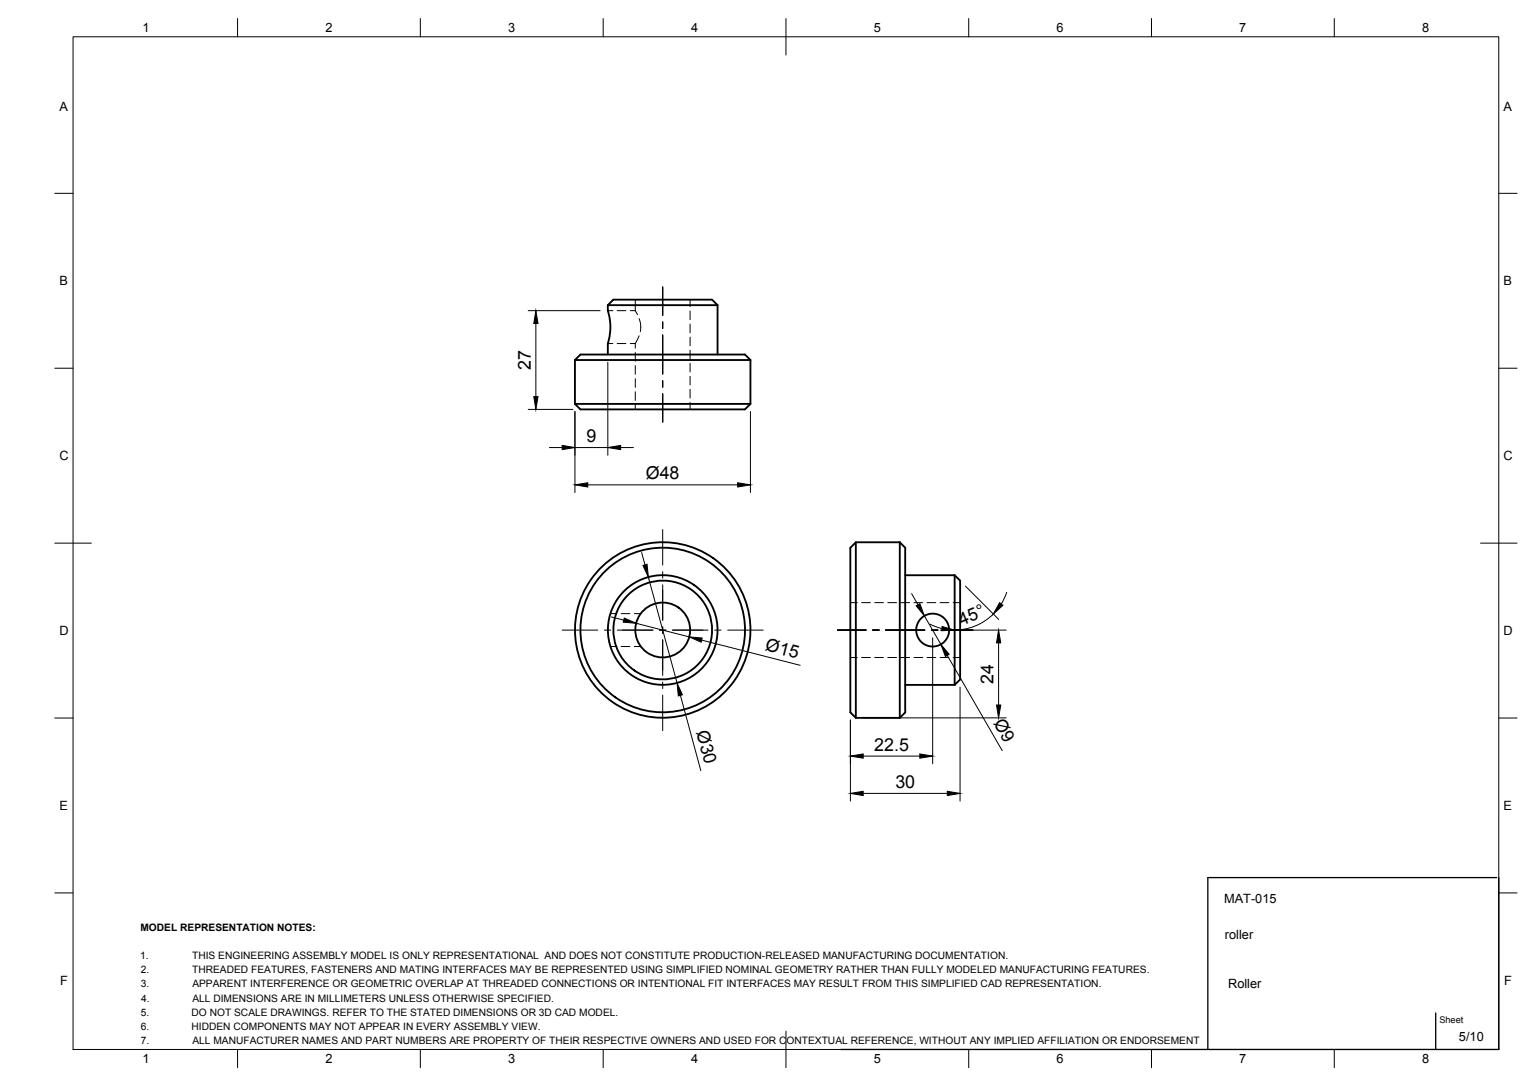
ISO-10303-21;
HEADER;
/* Generated by software containing ST-Developer
 * from STEP Tools, Inc. (www.steptools.com) 
 */

FILE_DESCRIPTION(
/* description */ ('STEP AP214'),
/* implementation_level */ '2;1');

FILE_NAME(
/* name */ 'Roller.step',
/* time_stamp */ '2026-11-14T06:03:18-08:00',
/* author */ (''),
/* organization */ (''),
/* preprocessor_version */ 'ST-DEVELOPER v20.2',
/* originating_system */ 'Autodesk Translation Framework v15.17.0.0',
/* authorisation */ '');

FILE_SCHEMA (('AUTOMOTIVE_DESIGN { 1 0 10303 214 3 1 1 }'));
ENDSEC;

DATA;
#10=MECHANICAL_DESIGN_GEOMETRIC_PRESENTATION_REPRESENTATION('',(#73),#3206);
#47=B_SPLINE_CURVE_WITH_KNOTS('',3,(#2691,#2692,#2693,#2694,#2695,#2696,
#2697,#2698,#2699,#2700,#2701,#2702,#2703,#2704,#2705,#2706,#2707,#2708),
 .UNSPECIFIED.,.F.,.F.,(4,2,2,2,2,2,2,2,4),(-1.36519473470625,-1.19451997041109,
-1.02384520611593,-0.853221286734528,-0.682597367353127,-0.511973447971726,
-0.341349528590325,-0.170674764295162,0.),.UNSPECIFIED.);
#48=B_SPLINE_CURVE_WITH_KNOTS('',3,(#2712,#2713,#2714,#2715,#2716,#2717,
#2718,#2719,#2720,#2721,#2722,#2723,#2724,#2725,#2726,#2727,#2728,#2729),
 .UNSPECIFIED.,.F.,.F.,(4,2,2,2,2,2,2,2,4),(-1.39899108486948,-1.22355122072177,
-1.04811135657406,-0.873803449504402,-0.699495542434742,-0.525187635365083,
-0.350879728295424,-0.175439864147712,0.),.UNSPECIFIED.);
#49=B_SPLINE_CURVE_WITH_KNOTS('',3,(#2730,#2731,#2732,#2733,#2734,#2735,
#2736,#2737,#2738,#2739,#2740,#2741,#2742,#2743,#2744,#2745,#2746,#2747),
 .UNSPECIFIED.,.F.,.F.,(4,2,2,2,2,2,2,2,4),(-2.79798216973897,-2.62254230559126,
-2.44710244144355,-2.27279453437389,-2.09848662730423,-1.92417872023457,
-1.74987081316491,-1.5744309490172,-1.39899108486948),.UNSPECIFIED.);
#50=B_SPLINE_CURVE_WITH_KNOTS('',3,(#2748,#2749,#2750,#2751,#2752,#2753,
#2754,#2755,#2756,#2757,#2758,#2759,#2760,#2761,#2762,#2763,#2764,#2765),
 .UNSPECIFIED.,.F.,.F.,(4,2,2,2,2,2,2,2,4),(0.,0.170674764295163,0.341349528590325,
0.511973447971726,0.682597367353127,0.853221286734528,1.02384520611593,
1.19451997041109,1.36519473470625),.UNSPECIFIED.);
#51=CONICAL_SURFACE('',#1904,13.5,0.785398163397445);
#52=CONICAL_SURFACE('',#1908,22.5,0.785398163397448);
#53=CONICAL_SURFACE('',#1912,24.,0.785398163397452);
#57=SHAPE_REPRESENTATION_RELATIONSHIP('SRR','None',#3240,#65);
#65=ADVANCED_BREP_SHAPE_REPRESENTATION('',(#81),#3199);
#73=STYLED_ITEM('',(#3288),#81);
#81=MANIFOLD_SOLID_BREP('Body1',#1780);
#95=PLANE('',#1922);
#96=PLANE('',#1923);
#97=PLANE('',#1924);
#150=FACE_BOUND('',#633,.T.);
#151=FACE_BOUND('',#635,.T.);
#152=FACE_BOUND('',#637,.T.);
#153=FACE_BOUND('',#639,.T.);
#154=FACE_BOUND('',#641,.T.);
#195=LINE('',#2672,#340);
#196=LINE('',#2680,#341);
#197=LINE('',#2686,#342);
#198=LINE('',#2710,#343);
#199=LINE('',#2767,#344);
#200=LINE('',#2772,#345);
#201=LINE('',#2776,#346);
#340=VECTOR('',#2144,13.5);
#341=VECTOR('',#2153,22.5);
#342=VECTOR('',#2160,24.);
#343=VECTOR('',#2165,4.5);
#344=VECTOR('',#2168,24.);
#345=VECTOR('',#2173,7.5);
#346=VECTOR('',#2178,15.);
#481=CYLINDRICAL_SURFACE('',#1915,4.5);
#482=CYLINDRICAL_SURFACE('',#1916,24.);
#483=CYLINDRICAL_SURFACE('',#1917,7.5);
#484=CYLINDRICAL_SURFACE('',#1920,15.);
#524=FACE_OUTER_BOUND('',#627,.T.);
#525=FACE_OUTER_BOUND('',#628,.T.);
#526=FACE_OUTER_BOUND('',#629,.T.);
#527=FACE_OUTER_BOUND('',#630,.T.);
#528=FACE_OUTER_BOUND('',#631,.T.);
#529=FACE_OUTER_BOUND('',#632,.T.);
#530=FACE_OUTER_BOUND('',#634,.T.);
#531=FACE_OUTER_BOUND('',#636,.T.);
#532=FACE_OUTER_BOUND('',#638,.T.);
#533=FACE_OUTER_BOUND('',#640,.T.);
#627=EDGE_LOOP('',(#1257,#1258,#1259,#1260,#1261));
#628=EDGE_LOOP('',(#1262,#1263,#1264,#1265,#1266));
#629=EDGE_LOOP('',(#1267,#1268,#1269,#1270));
#630=EDGE_LOOP('',(#1271,#1272,#1273,#1274,#1275,#1276));
#631=EDGE_LOOP('',(#1277,#1278,#1279,#1280,#1281));
#632=EDGE_LOOP('',(#1282,#1283,#1284,#1285));
#633=EDGE_LOOP('',(#1286,#1287));
#634=EDGE_LOOP('',(#1288,#1289,#1290,#1291,#1292));
#635=EDGE_LOOP('',(#1293,#1294));
#636=EDGE_LOOP('',(#1295));
#637=EDGE_LOOP('',(#1296));
#638=EDGE_LOOP('',(#1297));
#639=EDGE_LOOP('',(#1298));
#640=EDGE_LOOP('',(#1299));
#641=EDGE_LOOP('',(#1300));
#766=CIRCLE('',#1905,15.);
#767=CIRCLE('',#1906,15.);
#768=CIRCLE('',#1907,13.5);
#769=CIRCLE('',#1909,24.);
#770=CIRCLE('',#1910,24.);
#771=CIRCLE('',#1911,22.5);
#772=CIRCLE('',#1913,24.);
#773=CIRCLE('',#1914,22.5);
#774=CIRCLE('',#1918,7.5);
#775=CIRCLE('',#1919,7.5);
#776=CIRCLE('',#1921,15.);
#847=VERTEX_POINT('',#2667);
#848=VERTEX_POINT('',#2668);
#849=VERTEX_POINT('',#2671);
#850=VERTEX_POINT('',#2675);
#851=VERTEX_POINT('',#2676);
#852=VERTEX_POINT('',#2679);
#853=VERTEX_POINT('',#2683);
#854=VERTEX_POINT('',#2685);
#855=VERTEX_POINT('',#2689);
#856=VERTEX_POINT('',#2690);
#857=VERTEX_POINT('',#2709);
#858=VERTEX_POINT('',#2711);
#859=VERTEX_POINT('',#2769);
#860=VERTEX_POINT('',#2771);
#861=VERTEX_POINT('',#2775);
#1007=EDGE_CURVE('',#847,#848,#766,.T.);
#1008=EDGE_CURVE('',#848,#847,#767,.T.);
#1009=EDGE_CURVE('',#848,#849,#195,.T.);
#1010=EDGE_CURVE('',#849,#849,#768,.T.);
#1011=EDGE_CURVE('',#850,#851,#769,.T.);
#1012=EDGE_CURVE('',#851,#850,#770,.T.);
#1013=EDGE_CURVE('',#851,#852,#196,.T.);
#1014=EDGE_CURVE('',#852,#852,#771,.T.);
#1015=EDGE_CURVE('',#853,#853,#772,.T.);
#1016=EDGE_CURVE('',#853,#854,#197,.T.);
#1017=EDGE_CURVE('',#854,#854,#773,.T.);
#1018=EDGE_CURVE('',#855,#856,#47,.T.);
#1019=EDGE_CURVE('',#856,#857,#198,.T.);
#1020=EDGE_CURVE('',#857,#858,#48,.T.);
#1021=EDGE_CURVE('',#858,#857,#49,.T.);
#1022=EDGE_CURVE('',#856,#855,#50,.T.);
#1023=EDGE_CURVE('',#850,#853,#199,.T.);
#1024=EDGE_CURVE('',#859,#859,#774,.T.);
#1025=EDGE_CURVE('',#859,#860,#200,.T.);
#1026=EDGE_CURVE('',#860,#860,#775,.T.);
#1027=EDGE_CURVE('',#847,#861,#201,.T.);
#1028=EDGE_CURVE('',#861,#861,#776,.T.);
#1257=ORIENTED_EDGE('',*,*,#1007,.F.);
#1258=ORIENTED_EDGE('',*,*,#1008,.F.);
#1259=ORIENTED_EDGE('',*,*,#1009,.T.);
#1260=ORIENTED_EDGE('',*,*,#1010,.F.);
#1261=ORIENTED_EDGE('',*,*,#1009,.F.);
#1262=ORIENTED_EDGE('',*,*,#1011,.F.);
#1263=ORIENTED_EDGE('',*,*,#1012,.F.);
#1264=ORIENTED_EDGE('',*,*,#1013,.T.);
#1265=ORIENTED_EDGE('',*,*,#1014,.F.);
#1266=ORIENTED_EDGE('',*,*,#1013,.F.);
#1267=ORIENTED_EDGE('',*,*,#1015,.F.);
#1268=ORIENTED_EDGE('',*,*,#1016,.T.);
#1269=ORIENTED_EDGE('',*,*,#1017,.F.);
#1270=ORIENTED_EDGE('',*,*,#1016,.F.);
#1271=ORIENTED_EDGE('',*,*,#1018,.T.);
#1272=ORIENTED_EDGE('',*,*,#1019,.T.);
#1273=ORIENTED_EDGE('',*,*,#1020,.T.);
#1274=ORIENTED_EDGE('',*,*,#1021,.T.);
#1275=ORIENTED_EDGE('',*,*,#1019,.F.);
#1276=ORIENTED_EDGE('',*,*,#1022,.T.);
#1277=ORIENTED_EDGE('',*,*,#1011,.T.);
#1278=ORIENTED_EDGE('',*,*,#1012,.T.);
#1279=ORIENTED_EDGE('',*,*,#1023,.T.);
#1280=ORIENTED_EDGE('',*,*,#1015,.T.);
#1281=ORIENTED_EDGE('',*,*,#1023,.F.);
#1282=ORIENTED_EDGE('',*,*,#1024,.F.);
#1283=ORIENTED_EDGE('',*,*,#1025,.T.);
#1284=ORIENTED_EDGE('',*,*,#1026,.T.);
#1285=ORIENTED_EDGE('',*,*,#1025,.F.);
#1286=ORIENTED_EDGE('',*,*,#1021,.F.);
#1287=ORIENTED_EDGE('',*,*,#1020,.F.);
#1288=ORIENTED_EDGE('',*,*,#1007,.T.);
#1289=ORIENTED_EDGE('',*,*,#1008,.T.);
#1290=ORIENTED_EDGE('',*,*,#1027,.T.);
#1291=ORIENTED_EDGE('',*,*,#1028,.T.);
#1292=ORIENTED_EDGE('',*,*,#1027,.F.);
#1293=ORIENTED_EDGE('',*,*,#1018,.F.);
#1294=ORIENTED_EDGE('',*,*,#1022,.F.);
#1295=ORIENTED_EDGE('',*,*,#1017,.T.);
#1296=ORIENTED_EDGE('',*,*,#1026,.F.);
#1297=ORIENTED_EDGE('',*,*,#1014,.T.);
#1298=ORIENTED_EDGE('',*,*,#1028,.F.);
#1299=ORIENTED_EDGE('',*,*,#1010,.T.);
#1300=ORIENTED_EDGE('',*,*,#1024,.T.);
#1691=ADVANCED_FACE('',(#524),#51,.T.);
#1692=ADVANCED_FACE('',(#525),#52,.T.);
#1693=ADVANCED_FACE('',(#526),#53,.T.);
#1694=ADVANCED_FACE('',(#527),#481,.F.);
#1695=ADVANCED_FACE('',(#528),#482,.T.);
#1696=ADVANCED_FACE('',(#529,#150),#483,.F.);
#1697=ADVANCED_FACE('',(#530,#151),#484,.T.);
#1698=ADVANCED_FACE('',(#531,#152),#95,.F.);
#1699=ADVANCED_FACE('',(#532,#153),#96,.F.);
#1700=ADVANCED_FACE('',(#533,#154),#97,.F.);
#1780=CLOSED_SHELL('',(#1691,#1692,#1693,#1694,#1695,#1696,#1697,#1698,
#1699,#1700));
#1903=AXIS2_PLACEMENT_3D('',#2665,#2136,#2137);
#1904=AXIS2_PLACEMENT_3D('',#2666,#2138,#2139);
#1905=AXIS2_PLACEMENT_3D('',#2669,#2140,#2141);
#1906=AXIS2_PLACEMENT_3D('',#2670,#2142,#2143);
#1907=AXIS2_PLACEMENT_3D('',#2673,#2145,#2146);
#1908=AXIS2_PLACEMENT_3D('',#2674,#2147,#2148);
#1909=AXIS2_PLACEMENT_3D('',#2677,#2149,#2150);
#1910=AXIS2_PLACEMENT_3D('',#2678,#2151,#2152);
#1911=AXIS2_PLACEMENT_3D('',#2681,#2154,#2155);
#1912=AXIS2_PLACEMENT_3D('',#2682,#2156,#2157);
#1913=AXIS2_PLACEMENT_3D('',#2684,#2158,#2159);
#1914=AXIS2_PLACEMENT_3D('',#2687,#2161,#2162);
#1915=AXIS2_PLACEMENT_3D('',#2688,#2163,#2164);
#1916=AXIS2_PLACEMENT_3D('',#2766,#2166,#2167);
#1917=AXIS2_PLACEMENT_3D('',#2768,#2169,#2170);
#1918=AXIS2_PLACEMENT_3D('',#2770,#2171,#2172);
#1919=AXIS2_PLACEMENT_3D('',#2773,#2174,#2175);
#1920=AXIS2_PLACEMENT_3D('',#2774,#2176,#2177);
#1921=AXIS2_PLACEMENT_3D('',#2777,#2179,#2180);
#1922=AXIS2_PLACEMENT_3D('',#2778,#2181,#2182);
#1923=AXIS2_PLACEMENT_3D('',#2779,#2183,#2184);
#1924=AXIS2_PLACEMENT_3D('',#2780,#2185,#2186);
#2136=DIRECTION('axis',(0.,0.,1.));
#2137=DIRECTION('refdir',(1.,0.,0.));
#2138=DIRECTION('center_axis',(1.,0.,0.));
#2139=DIRECTION('ref_axis',(0.,0.,-1.));
#2140=DIRECTION('center_axis',(1.,0.,0.));
#2141=DIRECTION('ref_axis',(0.,0.,-1.));
#2142=DIRECTION('center_axis',(1.,0.,0.));
#2143=DIRECTION('ref_axis',(0.,0.,-1.));
#2144=DIRECTION('',(-0.70710678118655,8.6595605623549E-17,-0.707106781186545));
#2145=DIRECTION('center_axis',(-1.,0.,0.));
#2146=DIRECTION('ref_axis',(0.,0.,-1.));
#2147=DIRECTION('center_axis',(1.,0.,0.));
#2148=DIRECTION('ref_axis',(0.,0.,-1.));
#2149=DIRECTION('center_axis',(1.,0.,0.));
#2150=DIRECTION('ref_axis',(0.,0.,-1.));
#2151=DIRECTION('center_axis',(1.,0.,0.));
#2152=DIRECTION('ref_axis',(0.,0.,-1.));
#2153=DIRECTION('',(-0.707106781186548,8.65956056235493E-17,-0.707106781186547));
#2154=DIRECTION('center_axis',(-1.,0.,0.));
#2155=DIRECTION('ref_axis',(0.,0.,-1.));
#2156=DIRECTION('center_axis',(-1.,0.,0.));
#2157=DIRECTION('ref_axis',(0.,0.,1.));
#2158=DIRECTION('center_axis',(-1.,0.,0.));
#2159=DIRECTION('ref_axis',(0.,0.,1.));
#2160=DIRECTION('',(0.707106781186545,8.65956056235496E-17,0.70710678118655));
#2161=DIRECTION('center_axis',(1.,0.,0.));
#2162=DIRECTION('ref_axis',(0.,0.,1.));
#2163=DIRECTION('center_axis',(0.,-1.,0.));
#2164=DIRECTION('ref_axis',(0.,0.,-1.));
#2165=DIRECTION('',(0.,-1.,0.));
#2166=DIRECTION('center_axis',(-1.,0.,0.));
#2167=DIRECTION('ref_axis',(0.,0.,1.));
#2168=DIRECTION('',(1.,0.,0.));
#2169=DIRECTION('center_axis',(1.,0.,0.));
#2170=DIRECTION('ref_axis',(0.,0.,-1.));
#2171=DIRECTION('center_axis',(1.,0.,0.));
#2172=DIRECTION('ref_axis',(0.,0.,-1.));
#2173=DIRECTION('',(1.,0.,0.));
#2174=DIRECTION('center_axis',(1.,0.,0.));
#2175=DIRECTION('ref_axis',(0.,0.,-1.));
#2176=DIRECTION('center_axis',(-1.,0.,0.));
#2177=DIRECTION('ref_axis',(0.,0.,1.));
#2178=DIRECTION('',(1.,0.,0.));
#2179=DIRECTION('center_axis',(-1.,0.,0.));
#2180=DIRECTION('ref_axis',(0.,0.,1.));
#2181=DIRECTION('center_axis',(-1.,0.,0.));
#2182=DIRECTION('ref_axis',(0.,0.,1.));
#2183=DIRECTION('center_axis',(1.,0.,0.));
#2184=DIRECTION('ref_axis',(0.,0.,-1.));
#2185=DIRECTION('center_axis',(1.,0.,0.));
#2186=DIRECTION('ref_axis',(0.,0.,-1.));
#2665=CARTESIAN_POINT('',(0.,0.,0.));
#2666=CARTESIAN_POINT('Origin',(-26.3399803187666,0.0567527576880167,-1.75047265224548E-6));
#2667=CARTESIAN_POINT('',(-24.8399803187666,0.0567527576880185,-15.0000017504727));
#2668=CARTESIAN_POINT('',(-24.8399803187666,0.0567527576880148,14.9999982495274));
#2669=CARTESIAN_POINT('Origin',(-24.8399803187666,0.0567527576880167,-1.75047265224548E-6));
#2670=CARTESIAN_POINT('Origin',(-24.8399803187666,0.0567527576880167,-1.75047265224548E-6));
#2671=CARTESIAN_POINT('',(-26.3399803187666,0.056752757688015,13.4999982495273));
#2672=CARTESIAN_POINT('',(-26.3399803187666,0.056752757688015,13.4999982495273));
#2673=CARTESIAN_POINT('Origin',(-26.3399803187666,0.0567527576880167,-1.75047265224548E-6));
#2674=CARTESIAN_POINT('Origin',(-11.3399803187666,0.0567527576880167,-1.75047265224548E-6));
#2675=CARTESIAN_POINT('',(-9.83998031876658,0.0567527576880196,-24.0000017504727));
#2676=CARTESIAN_POINT('',(-9.83998031876658,0.0567527576880137,23.9999982495274));
#2677=CARTESIAN_POINT('Origin',(-9.83998031876658,0.0567527576880167,-1.75047265224548E-6));
#2678=CARTESIAN_POINT('Origin',(-9.83998031876658,0.0567527576880167,-1.75047265224548E-6));
#2679=CARTESIAN_POINT('',(-11.3399803187666,0.0567527576880139,22.4999982495273));
#2680=CARTESIAN_POINT('',(-11.3399803187666,0.0567527576880139,22.4999982495273));
#2681=CARTESIAN_POINT('Origin',(-11.3399803187666,0.0567527576880167,-1.75047265224548E-6));
#2682=CARTESIAN_POINT('Origin',(2.16001968123339,0.0567527576880167,-1.75047265224548E-6));
#2683=CARTESIAN_POINT('',(2.16001968123339,0.0567527576880137,-24.0000017504727));
#2684=CARTESIAN_POINT('Origin',(2.16001968123339,0.0567527576880167,-1.75047265224548E-6));
#2685=CARTESIAN_POINT('',(3.6600196812334,0.0567527576880139,-22.5000017504726));
#2686=CARTESIAN_POINT('',(2.16001968123339,0.0567527576880137,-24.0000017504727));
#2687=CARTESIAN_POINT('Origin',(3.6600196812334,0.0567527576880167,-1.75047265224548E-6));
#2688=CARTESIAN_POINT('Origin',(-18.8399803187666,18.056752757688,-1.75047264877604E-6));
#2689=CARTESIAN_POINT('',(-18.8399803187666,14.3658407789422,-4.50000175047265));
#2690=CARTESIAN_POINT('',(-18.8399803187666,14.3658407789422,4.49999824952735));
#2691=CARTESIAN_POINT('Ctrl Pts',(-18.8399803187666,14.3658407789422,-4.50000175047265));
#2692=CARTESIAN_POINT('Ctrl Pts',(-19.4088961997505,14.3658407789422,-4.50000175047265));
#2693=CARTESIAN_POINT('Ctrl Pts',(-20.013141546909,14.4033218435503,-4.38558312462148));
#2694=CARTESIAN_POINT('Ctrl Pts',(-21.1206936253408,14.5360270992361,-3.92530183970913));
#2695=CARTESIAN_POINT('Ctrl Pts',(-21.6243333805236,14.6290540336233,-3.57960971939459));
#2696=CARTESIAN_POINT('Ctrl Pts',(-22.4194698323699,14.8016561969128,-2.78447326754827));
#2697=CARTESIAN_POINT('Ctrl Pts',(-22.7652536793161,14.8928206825392,-2.28078537898198));
#2698=CARTESIAN_POINT('Ctrl Pts',(-23.2256026885326,15.0212047585055,-1.17305832669546));
#2699=CARTESIAN_POINT('Ctrl Pts',(-23.3399803187666,15.056752757688,-0.568748148410651));
#2700=CARTESIAN_POINT('Ctrl Pts',(-23.3399803187666,15.056752757688,0.568744647465355));
#2701=CARTESIAN_POINT('Ctrl Pts',(-23.2256026885326,15.0212047585055,1.17305482575017));
#2702=CARTESIAN_POINT('Ctrl Pts',(-22.7652536793161,14.8928206825392,2.28078187803669));
#2703=CARTESIAN_POINT('Ctrl Pts',(-22.4194698323699,14.8016561969128,2.78446976660297));
#2704=CARTESIAN_POINT('Ctrl Pts',(-21.6243333805236,14.6290540336233,3.57960621844929));
#2705=CARTESIAN_POINT('Ctrl Pts',(-21.1206936253408,14.5360270992361,3.92529833876383));
#2706=CARTESIAN_POINT('Ctrl Pts',(-20.013141546909,14.4033218435503,4.38557962367618));
#2707=CARTESIAN_POINT('Ctrl Pts',(-19.4088961997505,14.3658407789422,4.49999824952735));
#2708=CARTESIAN_POINT('Ctrl Pts',(-18.8399803187666,14.3658407789422,4.49999824952735));
#2709=CARTESIAN_POINT('',(-18.8399803187666,6.05675275768802,4.49999824952735));
#2710=CARTESIAN_POINT('',(-18.8399803187666,18.056752757688,4.49999824952735));
#2711=CARTESIAN_POINT('',(-18.8399803187666,6.05675275768802,-4.50000175047266));
#2712=CARTESIAN_POINT('Ctrl Pts',(-18.8399803187666,6.05675275768802,4.49999824952735));
#2713=CARTESIAN_POINT('Ctrl Pts',(-19.4247798659256,6.05675275768802,4.49999824952735));
#2714=CARTESIAN_POINT('Ctrl Pts',(-20.0327174049161,6.15125943860946,4.37996991421688));
#2715=CARTESIAN_POINT('Ctrl Pts',(-21.1340415543933,6.45855603358751,3.91714882470871));
#2716=CARTESIAN_POINT('Ctrl Pts',(-21.6294259483511,6.66438066194848,3.57451365062178));
#2717=CARTESIAN_POINT('Ctrl Pts',(-22.4119630421001,7.03101594719294,2.79197655687281));
#2718=CARTESIAN_POINT('Ctrl Pts',(-22.7563617548165,7.21926420444051,2.29589436091356));
#2719=CARTESIAN_POINT('Ctrl Pts',(-23.220735898688,7.48336337711206,1.19086529875321));
#2720=CARTESIAN_POINT('Ctrl Pts',(-23.3399803187666,7.55675275768802,0.581024606426215));
#2721=CARTESIAN_POINT('Ctrl Pts',(-23.3399803187666,7.55675275768802,-0.581028107371513));
#2722=CARTESIAN_POINT('Ctrl Pts',(-23.220735898688,7.48336337711206,-1.19086879969851));
#2723=CARTESIAN_POINT('Ctrl Pts',(-22.7563617548165,7.21926420444051,-2.29589786185886));
#2724=CARTESIAN_POINT('Ctrl Pts',(-22.4119630421001,7.03101594719294,-2.79198005781811));
#2725=CARTESIAN_POINT('Ctrl Pts',(-21.6294259483511,6.66438066194849,-3.57451715156708));
#2726=CARTESIAN_POINT('Ctrl Pts',(-21.1340415543933,6.45855603358751,-3.91715232565401));
#2727=CARTESIAN_POINT('Ctrl Pts',(-20.0327174049161,6.15125943860947,-4.37997341516218));
#2728=CARTESIAN_POINT('Ctrl Pts',(-19.4247798659256,6.05675275768802,-4.50000175047265));
#2729=CARTESIAN_POINT('Ctrl Pts',(-18.8399803187666,6.05675275768802,-4.50000175047265));
#2730=CARTESIAN_POINT('Ctrl Pts',(-18.8399803187666,6.05675275768802,-4.50000175047265));
#2731=CARTESIAN_POINT('Ctrl Pts',(-18.2551807716076,6.05675275768802,-4.50000175047265));
#2732=CARTESIAN_POINT('Ctrl Pts',(-17.6472432326171,6.15125943860946,-4.37997341516218));
#2733=CARTESIAN_POINT('Ctrl Pts',(-16.5459190831399,6.45855603358751,-3.91715232565401));
#2734=CARTESIAN_POINT('Ctrl Pts',(-16.0505346891821,6.66438066194849,-3.57451715156707));
#2735=CARTESIAN_POINT('Ctrl Pts',(-15.2679975954331,7.03101594719294,-2.79198005781811));
#2736=CARTESIAN_POINT('Ctrl Pts',(-14.9235988827167,7.21926420444051,-2.29589786185886));
#2737=CARTESIAN_POINT('Ctrl Pts',(-14.4592247388452,7.48336337711206,-1.1908687996985));
#2738=CARTESIAN_POINT('Ctrl Pts',(-14.3399803187666,7.55675275768802,-0.581028107371512));
#2739=CARTESIAN_POINT('Ctrl Pts',(-14.3399803187666,7.55675275768802,0.581024606426216));
#2740=CARTESIAN_POINT('Ctrl Pts',(-14.4592247388452,7.48336337711206,1.19086529875321));
#2741=CARTESIAN_POINT('Ctrl Pts',(-14.9235988827167,7.21926420444051,2.29589436091356));
#2742=CARTESIAN_POINT('Ctrl Pts',(-15.2679975954331,7.03101594719294,2.79197655687282));
#2743=CARTESIAN_POINT('Ctrl Pts',(-16.0505346891821,6.66438066194848,3.57451365062178));
#2744=CARTESIAN_POINT('Ctrl Pts',(-16.5459190831399,6.45855603358751,3.91714882470872));
#2745=CARTESIAN_POINT('Ctrl Pts',(-17.6472432326171,6.15125943860946,4.37996991421688));
#2746=CARTESIAN_POINT('Ctrl Pts',(-18.2551807716076,6.05675275768802,4.49999824952735));
#2747=CARTESIAN_POINT('Ctrl Pts',(-18.8399803187666,6.05675275768802,4.49999824952735));
#2748=CARTESIAN_POINT('Ctrl Pts',(-18.8399803187666,14.3658407789422,4.49999824952735));
#2749=CARTESIAN_POINT('Ctrl Pts',(-18.2710644377827,14.3658407789422,4.49999824952735));
#2750=CARTESIAN_POINT('Ctrl Pts',(-17.6668190906242,14.4033218435503,4.38557962367618));
#2751=CARTESIAN_POINT('Ctrl Pts',(-16.5592670121924,14.5360270992361,3.92529833876383));
#2752=CARTESIAN_POINT('Ctrl Pts',(-16.0556272570096,14.6290540336233,3.57960621844929));
#2753=CARTESIAN_POINT('Ctrl Pts',(-15.2604908051633,14.8016561969128,2.78446976660297));
#2754=CARTESIAN_POINT('Ctrl Pts',(-14.9147069582171,14.8928206825392,2.28078187803668));
#2755=CARTESIAN_POINT('Ctrl Pts',(-14.4543579490006,15.0212047585055,1.17305482575016));
#2756=CARTESIAN_POINT('Ctrl Pts',(-14.3399803187666,15.056752757688,0.568744647465353));
#2757=CARTESIAN_POINT('Ctrl Pts',(-14.3399803187666,15.056752757688,-0.568748148410654));
#2758=CARTESIAN_POINT('Ctrl Pts',(-14.4543579490006,15.0212047585055,-1.17305832669547));
#2759=CARTESIAN_POINT('Ctrl Pts',(-14.9147069582171,14.8928206825392,-2.28078537898199));
#2760=CARTESIAN_POINT('Ctrl Pts',(-15.2604908051633,14.8016561969128,-2.78447326754827));
#2761=CARTESIAN_POINT('Ctrl Pts',(-16.0556272570096,14.6290540336233,-3.57960971939459));
#2762=CARTESIAN_POINT('Ctrl Pts',(-16.5592670121924,14.5360270992361,-3.92530183970913));
#2763=CARTESIAN_POINT('Ctrl Pts',(-17.6668190906242,14.4033218435503,-4.38558312462147));
#2764=CARTESIAN_POINT('Ctrl Pts',(-18.2710644377827,14.3658407789422,-4.50000175047265));
#2765=CARTESIAN_POINT('Ctrl Pts',(-18.8399803187666,14.3658407789422,-4.50000175047265));
#2766=CARTESIAN_POINT('Origin',(-26.3399803187666,0.0567527576880167,-1.75047265224548E-6));
#2767=CARTESIAN_POINT('',(-26.3399803187666,0.0567527576880137,-24.0000017504727));
#2768=CARTESIAN_POINT('Origin',(-27.8399803187666,0.0567527576880167,-1.75047265224548E-6));
#2769=CARTESIAN_POINT('',(-26.3399803187666,0.0567527576880158,7.49999824952735));
#2770=CARTESIAN_POINT('Origin',(-26.3399803187666,0.0567527576880167,-1.75047265224548E-6));
#2771=CARTESIAN_POINT('',(3.6600196812334,0.0567527576880158,7.49999824952735));
#2772=CARTESIAN_POINT('',(-27.8399803187666,0.0567527576880158,7.49999824952735));
#2773=CARTESIAN_POINT('Origin',(3.6600196812334,0.0567527576880167,-1.75047265224548E-6));
#2774=CARTESIAN_POINT('Origin',(-26.3399803187666,0.0567527576880167,-1.75047265224548E-6));
#2775=CARTESIAN_POINT('',(-11.3399803187666,0.0567527576880148,-15.0000017504727));
#2776=CARTESIAN_POINT('',(-26.3399803187666,0.0567527576880148,-15.0000017504727));
#2777=CARTESIAN_POINT('Origin',(-11.3399803187666,0.0567527576880167,-1.75047265224548E-6));
#2778=CARTESIAN_POINT('Origin',(3.6600196812334,0.0567527576880167,-1.75047265224548E-6));
#2779=CARTESIAN_POINT('Origin',(-11.3399803187666,24.056752757688,-1.75047264877604E-6));
#2780=CARTESIAN_POINT('Origin',(-26.3399803187666,15.056752757688,-1.75047265571493E-6));
#3189=UNCERTAINTY_MEASURE_WITH_UNIT(LENGTH_MEASURE(0.01),#3207,
'DISTANCE_ACCURACY_VALUE',
'Maximum model space distance between geometric entities at asserted c
onnectivities');
#3196=UNCERTAINTY_MEASURE_WITH_UNIT(LENGTH_MEASURE(0.01),#3207,
'DISTANCE_ACCURACY_VALUE',
'Maximum model space distance between geometric entities at asserted c
onnectivities');
#3199=(
GEOMETRIC_REPRESENTATION_CONTEXT(3)
GLOBAL_UNCERTAINTY_ASSIGNED_CONTEXT((#3189))
GLOBAL_UNIT_ASSIGNED_CONTEXT((#3207,#3209,#3210))
REPRESENTATION_CONTEXT('','3D')
);
#3206=(
GEOMETRIC_REPRESENTATION_CONTEXT(3)
GLOBAL_UNCERTAINTY_ASSIGNED_CONTEXT((#3196))
GLOBAL_UNIT_ASSIGNED_CONTEXT((#3207,#3209,#3210))
REPRESENTATION_CONTEXT('','3D')
);
#3207=(
LENGTH_UNIT()
NAMED_UNIT(*)
SI_UNIT(.MILLI.,.METRE.)
);
#3209=(
NAMED_UNIT(*)
PLANE_ANGLE_UNIT()
SI_UNIT($,.RADIAN.)
);
#3210=(
NAMED_UNIT(*)
SI_UNIT($,.STERADIAN.)
SOLID_ANGLE_UNIT()
);
#3213=SHAPE_DEFINITION_REPRESENTATION(#3222,#3240);
#3222=PRODUCT_DEFINITION_SHAPE('',$,#3250);
#3240=SHAPE_REPRESENTATION('',(#1903),#3199);
#3247=PRODUCT_DEFINITION_CONTEXT('part definition',#3276,'design');
#3250=PRODUCT_DEFINITION('roller','Roller',#3259,#3247);
#3259=PRODUCT_DEFINITION_FORMATION('',$,#3280);
#3276=APPLICATION_CONTEXT(
'Core Data for Automotive Mechanical Design Process');
#3277=PRODUCT_CONTEXT('part definition',#3276,'mechanical');
#3280=PRODUCT('roller','Roller',$,(#3277));
#3288=PRESENTATION_STYLE_ASSIGNMENT((#3292));
#3292=SURFACE_STYLE_USAGE(.BOTH.,#3296);
#3296=SURFACE_SIDE_STYLE('',(#3300));
#3300=SURFACE_STYLE_FILL_AREA(#3304);
#3304=FILL_AREA_STYLE('Opaque(61,176,222)',(#3308));
#3308=FILL_AREA_STYLE_COLOUR('Opaque(61,176,222)',#3312);
#3312=COLOUR_RGB('Opaque(61,176,222)',0.23921568627451,0.690196078431373,
0.870588235294118);
ENDSEC;
END-ISO-10303-21;
